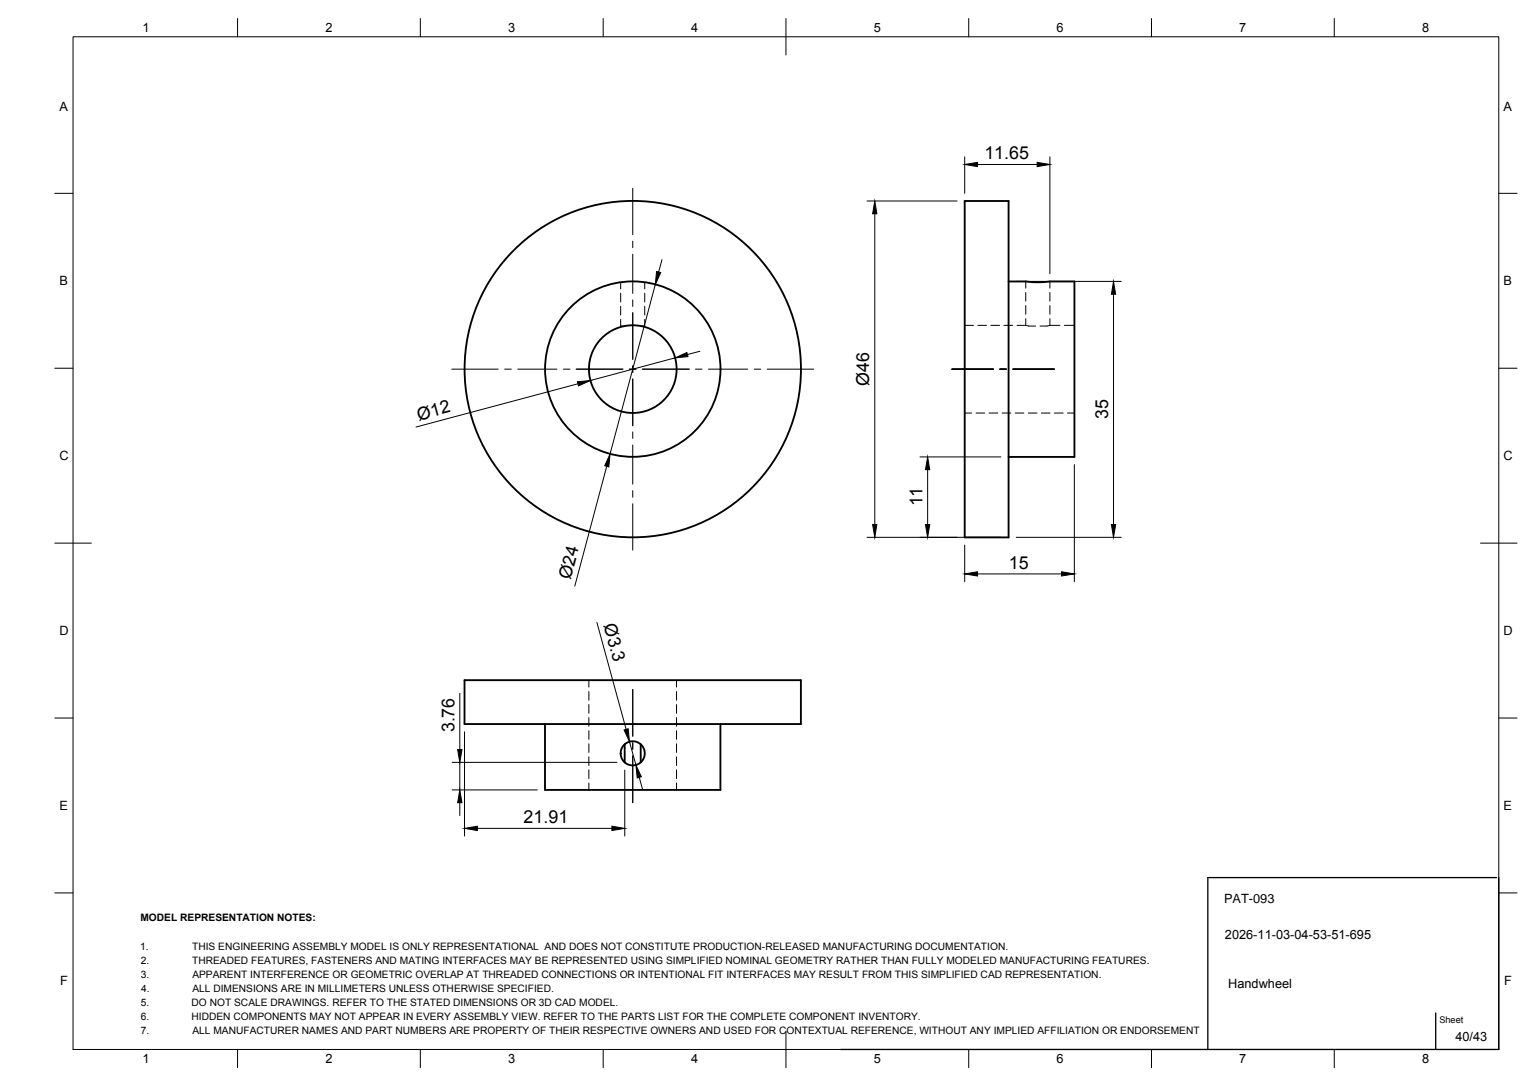
ISO-10303-21;
HEADER;
/* Generated by software containing ST-Developer
 * from STEP Tools, Inc. (www.steptools.com) 
 */

FILE_DESCRIPTION(
/* description */ ('Self-centering screw clamp'),
/* implementation_level */ '2;1');

FILE_NAME(
/* name */ 'Handwheel.step',
/* time_stamp */ '2026-10-28T03:25:31-07:00',
/* author */ (''),
/* organization */ (''),
/* preprocessor_version */ 'ST-DEVELOPER v20.2',
/* originating_system */ 'Autodesk Translation Framework v15.17.0.0',
/* authorisation */ '');

FILE_SCHEMA (('AUTOMOTIVE_DESIGN { 1 0 10303 214 3 1 1 }'));
ENDSEC;

DATA;
#10=MECHANICAL_DESIGN_GEOMETRIC_PRESENTATION_REPRESENTATION('',(#666),#16799);
#528=B_SPLINE_CURVE_WITH_KNOTS('',3,(#16250,#16251,#16252,#16253,#16254,
#16255),.UNSPECIFIED.,.F.,.F.,(4,2,4),(0.635430324955929,0.687528937234027,
0.750024497760672),.UNSPECIFIED.);
#529=B_SPLINE_CURVE_WITH_KNOTS('',3,(#16259,#16260,#16261,#16262,#16263,
#16264),.UNSPECIFIED.,.F.,.F.,(4,2,4),(0.250008165920224,0.312503726446869,
0.364602338724964),.UNSPECIFIED.);
#530=B_SPLINE_CURVE_WITH_KNOTS('',3,(#16265,#16266,#16267,#16268,#16269,
#16270),.UNSPECIFIED.,.F.,.F.,(4,2,4),(0.135413993115483,0.187512605393579,
0.250008165920224),.UNSPECIFIED.);
#531=B_SPLINE_CURVE_WITH_KNOTS('',3,(#16271,#16272,#16273,#16274,#16275,
#16276),.UNSPECIFIED.,.F.,.F.,(4,2,4),(0.750024497760672,0.812520058287317,
0.864618670565415),.UNSPECIFIED.);
#532=B_SPLINE_CURVE_WITH_KNOTS('',3,(#16280,#16281,#16282,#16283,#16284,
#16285,#16286,#16287,#16288,#16289),.UNSPECIFIED.,.F.,.F.,(4,2,2,2,4),(0.,
0.0622384309821294,0.124476861964259,0.186714529331343,0.248952196698427),
 .UNSPECIFIED.);
#533=B_SPLINE_CURVE_WITH_KNOTS('',3,(#16291,#16292,#16293,#16294,#16295,
#16296,#16297,#16298,#16299,#16300),.UNSPECIFIED.,.F.,.F.,(4,2,2,2,4),(0.74685659009528,
0.809094257462364,0.871331924829448,0.933570355811577,0.995808786793707),
 .UNSPECIFIED.);
#534=B_SPLINE_CURVE_WITH_KNOTS('',3,(#16301,#16302,#16303,#16304,#16305,
#16306,#16307,#16308,#16309,#16310,#16311,#16312,#16313,#16314,#16315,#16316,
#16317,#16318),.UNSPECIFIED.,.F.,.F.,(4,2,2,2,2,2,2,2,4),(0.248952196698427,
0.311189864065511,0.373427531432595,0.435665962414724,0.497904393396853,
0.560142824378983,0.622381255361112,0.684618922728196,0.74685659009528),
 .UNSPECIFIED.);
#577=SHAPE_REPRESENTATION_RELATIONSHIP('SRR','None',#17055,#618);
#618=ADVANCED_BREP_SHAPE_REPRESENTATION('',(#713),#16793);
#666=STYLED_ITEM('',(#17319),#713);
#713=MANIFOLD_SOLID_BREP('Body1',#9118);
#1003=FACE_BOUND('',#2518,.T.);
#1004=FACE_BOUND('',#2522,.T.);
#1005=FACE_BOUND('',#2524,.T.);
#1240=PLANE('',#10557);
#1241=PLANE('',#10561);
#1242=PLANE('',#10562);
#1243=PLANE('',#10569);
#1244=PLANE('',#10570);
#1724=FACE_OUTER_BOUND('',#2513,.T.);
#1725=FACE_OUTER_BOUND('',#2514,.T.);
#1726=FACE_OUTER_BOUND('',#2515,.T.);
#1727=FACE_OUTER_BOUND('',#2516,.T.);
#1728=FACE_OUTER_BOUND('',#2517,.T.);
#1729=FACE_OUTER_BOUND('',#2519,.T.);
#1730=FACE_OUTER_BOUND('',#2520,.T.);
#1731=FACE_OUTER_BOUND('',#2521,.T.);
#1732=FACE_OUTER_BOUND('',#2523,.T.);
#2513=EDGE_LOOP('',(#8133,#8134,#8135,#8136));
#2514=EDGE_LOOP('',(#8137,#8138));
#2515=EDGE_LOOP('',(#8139,#8140,#8141,#8142,#8143,#8144,#8145,#8146,#8147,
#8148,#8149));
#2516=EDGE_LOOP('',(#8150,#8151));
#2517=EDGE_LOOP('',(#8152));
#2518=EDGE_LOOP('',(#8153));
#2519=EDGE_LOOP('',(#8154,#8155,#8156,#8157,#8158,#8159,#8160,#8161,#8162,
#8163,#8164,#8165));
#2520=EDGE_LOOP('',(#8166,#8167,#8168,#8169,#8170,#8171,#8172,#8173,#8174));
#2521=EDGE_LOOP('',(#8175));
#2522=EDGE_LOOP('',(#8176));
#2523=EDGE_LOOP('',(#8177));
#2524=EDGE_LOOP('',(#8178));
#3086=LINE('',#16240,#3659);
#3087=LINE('',#16245,#3660);
#3088=LINE('',#16278,#3661);
#3089=LINE('',#16320,#3662);
#3090=LINE('',#16327,#3663);
#3091=LINE('',#16329,#3664);
#3092=LINE('',#16334,#3665);
#3093=LINE('',#16335,#3666);
#3659=VECTOR('',#13219,2.3);
#3660=VECTOR('',#13224,1.);
#3661=VECTOR('',#13231,0.164999999999999);
#3662=VECTOR('',#13234,1.);
#3663=VECTOR('',#13243,0.6);
#3664=VECTOR('',#13244,0.6);
#3665=VECTOR('',#13251,1.2);
#3666=VECTOR('',#13252,1.2);
#4199=CIRCLE('',#10555,2.3);
#4200=CIRCLE('',#10556,2.3);
#4201=CIRCLE('',#10558,0.164999999999999);
#4202=CIRCLE('',#10560,0.164999999999999);
#4203=CIRCLE('',#10563,1.2);
#4204=CIRCLE('',#10565,0.6);
#4205=CIRCLE('',#10566,0.6);
#4206=CIRCLE('',#10568,1.2);
#4904=VERTEX_POINT('',#16237);
#4905=VERTEX_POINT('',#16239);
#4906=VERTEX_POINT('',#16243);
#4907=VERTEX_POINT('',#16244);
#4908=VERTEX_POINT('',#16248);
#4909=VERTEX_POINT('',#16249);
#4910=VERTEX_POINT('',#16256);
#4911=VERTEX_POINT('',#16258);
#4912=VERTEX_POINT('',#16277);
#4913=VERTEX_POINT('',#16279);
#4914=VERTEX_POINT('',#16290);
#4915=VERTEX_POINT('',#16322);
#4916=VERTEX_POINT('',#16325);
#4917=VERTEX_POINT('',#16328);
#4918=VERTEX_POINT('',#16332);
#5991=EDGE_CURVE('',#4904,#4904,#4199,.T.);
#5992=EDGE_CURVE('',#4904,#4905,#3086,.T.);
#5993=EDGE_CURVE('',#4905,#4905,#4200,.T.);
#5994=EDGE_CURVE('',#4906,#4907,#3087,.T.);
#5995=EDGE_CURVE('',#4906,#4907,#4201,.T.);
#5996=EDGE_CURVE('',#4908,#4909,#528,.T.);
#5997=EDGE_CURVE('',#4910,#4908,#4202,.T.);
#5998=EDGE_CURVE('',#4911,#4910,#529,.T.);
#5999=EDGE_CURVE('',#4907,#4911,#530,.T.);
#6000=EDGE_CURVE('',#4909,#4906,#531,.T.);
#6001=EDGE_CURVE('',#4909,#4912,#3088,.T.);
#6002=EDGE_CURVE('',#4913,#4912,#532,.T.);
#6003=EDGE_CURVE('',#4914,#4913,#533,.T.);
#6004=EDGE_CURVE('',#4912,#4914,#534,.T.);
#6005=EDGE_CURVE('',#4910,#4908,#3089,.T.);
#6006=EDGE_CURVE('',#4915,#4915,#4203,.T.);
#6007=EDGE_CURVE('',#4916,#4916,#4204,.T.);
#6008=EDGE_CURVE('',#4916,#4911,#3090,.T.);
#6009=EDGE_CURVE('',#4909,#4917,#3091,.T.);
#6010=EDGE_CURVE('',#4917,#4917,#4205,.T.);
#6011=EDGE_CURVE('',#4918,#4918,#4206,.T.);
#6012=EDGE_CURVE('',#4918,#4914,#3092,.T.);
#6013=EDGE_CURVE('',#4912,#4915,#3093,.T.);
#8133=ORIENTED_EDGE('',*,*,#5991,.F.);
#8134=ORIENTED_EDGE('',*,*,#5992,.T.);
#8135=ORIENTED_EDGE('',*,*,#5993,.F.);
#8136=ORIENTED_EDGE('',*,*,#5992,.F.);
#8137=ORIENTED_EDGE('',*,*,#5994,.F.);
#8138=ORIENTED_EDGE('',*,*,#5995,.T.);
#8139=ORIENTED_EDGE('',*,*,#5996,.F.);
#8140=ORIENTED_EDGE('',*,*,#5997,.F.);
#8141=ORIENTED_EDGE('',*,*,#5998,.F.);
#8142=ORIENTED_EDGE('',*,*,#5999,.F.);
#8143=ORIENTED_EDGE('',*,*,#5995,.F.);
#8144=ORIENTED_EDGE('',*,*,#6000,.F.);
#8145=ORIENTED_EDGE('',*,*,#6001,.T.);
#8146=ORIENTED_EDGE('',*,*,#6002,.F.);
#8147=ORIENTED_EDGE('',*,*,#6003,.F.);
#8148=ORIENTED_EDGE('',*,*,#6004,.F.);
#8149=ORIENTED_EDGE('',*,*,#6001,.F.);
#8150=ORIENTED_EDGE('',*,*,#6005,.F.);
#8151=ORIENTED_EDGE('',*,*,#5997,.T.);
#8152=ORIENTED_EDGE('',*,*,#5993,.T.);
#8153=ORIENTED_EDGE('',*,*,#6006,.F.);
#8154=ORIENTED_EDGE('',*,*,#6007,.F.);
#8155=ORIENTED_EDGE('',*,*,#6008,.T.);
#8156=ORIENTED_EDGE('',*,*,#5998,.T.);
#8157=ORIENTED_EDGE('',*,*,#6005,.T.);
#8158=ORIENTED_EDGE('',*,*,#5996,.T.);
#8159=ORIENTED_EDGE('',*,*,#6009,.T.);
#8160=ORIENTED_EDGE('',*,*,#6010,.T.);
#8161=ORIENTED_EDGE('',*,*,#6009,.F.);
#8162=ORIENTED_EDGE('',*,*,#6000,.T.);
#8163=ORIENTED_EDGE('',*,*,#5994,.T.);
#8164=ORIENTED_EDGE('',*,*,#5999,.T.);
#8165=ORIENTED_EDGE('',*,*,#6008,.F.);
#8166=ORIENTED_EDGE('',*,*,#6011,.F.);
#8167=ORIENTED_EDGE('',*,*,#6012,.T.);
#8168=ORIENTED_EDGE('',*,*,#6003,.T.);
#8169=ORIENTED_EDGE('',*,*,#6002,.T.);
#8170=ORIENTED_EDGE('',*,*,#6013,.T.);
#8171=ORIENTED_EDGE('',*,*,#6006,.T.);
#8172=ORIENTED_EDGE('',*,*,#6013,.F.);
#8173=ORIENTED_EDGE('',*,*,#6004,.T.);
#8174=ORIENTED_EDGE('',*,*,#6012,.F.);
#8175=ORIENTED_EDGE('',*,*,#6011,.T.);
#8176=ORIENTED_EDGE('',*,*,#6007,.T.);
#8177=ORIENTED_EDGE('',*,*,#5991,.T.);
#8178=ORIENTED_EDGE('',*,*,#6010,.F.);
#8557=CYLINDRICAL_SURFACE('',#10554,2.3);
#8558=CYLINDRICAL_SURFACE('',#10559,0.164999999999999);
#8559=CYLINDRICAL_SURFACE('',#10564,0.6);
#8560=CYLINDRICAL_SURFACE('',#10567,1.2);
#9022=ADVANCED_FACE('',(#1724),#8557,.T.);
#9023=ADVANCED_FACE('',(#1725),#1240,.T.);
#9024=ADVANCED_FACE('',(#1726),#8558,.F.);
#9025=ADVANCED_FACE('',(#1727),#1241,.T.);
#9026=ADVANCED_FACE('',(#1728,#1003),#1242,.T.);
#9027=ADVANCED_FACE('',(#1729),#8559,.F.);
#9028=ADVANCED_FACE('',(#1730),#8560,.T.);
#9029=ADVANCED_FACE('',(#1731,#1004),#1243,.T.);
#9030=ADVANCED_FACE('',(#1732,#1005),#1244,.F.);
#9118=CLOSED_SHELL('',(#9022,#9023,#9024,#9025,#9026,#9027,#9028,#9029,
#9030));
#10553=AXIS2_PLACEMENT_3D('',#16235,#13213,#13214);
#10554=AXIS2_PLACEMENT_3D('',#16236,#13215,#13216);
#10555=AXIS2_PLACEMENT_3D('',#16238,#13217,#13218);
#10556=AXIS2_PLACEMENT_3D('',#16241,#13220,#13221);
#10557=AXIS2_PLACEMENT_3D('',#16242,#13222,#13223);
#10558=AXIS2_PLACEMENT_3D('',#16246,#13225,#13226);
#10559=AXIS2_PLACEMENT_3D('',#16247,#13227,#13228);
#10560=AXIS2_PLACEMENT_3D('',#16257,#13229,#13230);
#10561=AXIS2_PLACEMENT_3D('',#16319,#13232,#13233);
#10562=AXIS2_PLACEMENT_3D('',#16321,#13235,#13236);
#10563=AXIS2_PLACEMENT_3D('',#16323,#13237,#13238);
#10564=AXIS2_PLACEMENT_3D('',#16324,#13239,#13240);
#10565=AXIS2_PLACEMENT_3D('',#16326,#13241,#13242);
#10566=AXIS2_PLACEMENT_3D('',#16330,#13245,#13246);
#10567=AXIS2_PLACEMENT_3D('',#16331,#13247,#13248);
#10568=AXIS2_PLACEMENT_3D('',#16333,#13249,#13250);
#10569=AXIS2_PLACEMENT_3D('',#16336,#13253,#13254);
#10570=AXIS2_PLACEMENT_3D('',#16337,#13255,#13256);
#13213=DIRECTION('axis',(0.,0.,1.));
#13214=DIRECTION('refdir',(1.,0.,0.));
#13215=DIRECTION('center_axis',(1.,0.,0.));
#13216=DIRECTION('ref_axis',(0.,0.,-1.));
#13217=DIRECTION('center_axis',(-1.,0.,0.));
#13218=DIRECTION('ref_axis',(0.,0.,-1.));
#13219=DIRECTION('',(1.,0.,0.));
#13220=DIRECTION('center_axis',(1.,0.,0.));
#13221=DIRECTION('ref_axis',(0.,0.,-1.));
#13222=DIRECTION('center_axis',(0.,0.,1.));
#13223=DIRECTION('ref_axis',(1.,0.,0.));
#13224=DIRECTION('',(1.,0.,0.));
#13225=DIRECTION('center_axis',(0.,0.,1.));
#13226=DIRECTION('ref_axis',(1.,0.,0.));
#13227=DIRECTION('center_axis',(0.,0.,1.));
#13228=DIRECTION('ref_axis',(1.,0.,0.));
#13229=DIRECTION('center_axis',(0.,0.,1.));
#13230=DIRECTION('ref_axis',(1.,0.,0.));
#13231=DIRECTION('',(0.,0.,1.));
#13232=DIRECTION('center_axis',(0.,0.,1.));
#13233=DIRECTION('ref_axis',(1.,0.,0.));
#13234=DIRECTION('',(-1.,0.,0.));
#13235=DIRECTION('center_axis',(1.,0.,0.));
#13236=DIRECTION('ref_axis',(0.,0.,-1.));
#13237=DIRECTION('center_axis',(1.,0.,0.));
#13238=DIRECTION('ref_axis',(0.,0.,-1.));
#13239=DIRECTION('center_axis',(1.,0.,0.));
#13240=DIRECTION('ref_axis',(0.,0.,-1.));
#13241=DIRECTION('center_axis',(-1.,0.,0.));
#13242=DIRECTION('ref_axis',(0.,0.,-1.));
#13243=DIRECTION('',(-1.,0.,0.));
#13244=DIRECTION('',(-1.,0.,0.));
#13245=DIRECTION('center_axis',(-1.,0.,0.));
#13246=DIRECTION('ref_axis',(0.,0.,-1.));
#13247=DIRECTION('center_axis',(1.,0.,0.));
#13248=DIRECTION('ref_axis',(0.,0.,-1.));
#13249=DIRECTION('center_axis',(1.,0.,0.));
#13250=DIRECTION('ref_axis',(0.,0.,-1.));
#13251=DIRECTION('',(-1.,0.,0.));
#13252=DIRECTION('',(-1.,0.,0.));
#13253=DIRECTION('center_axis',(1.,0.,0.));
#13254=DIRECTION('ref_axis',(0.,0.,-1.));
#13255=DIRECTION('center_axis',(1.,0.,0.));
#13256=DIRECTION('ref_axis',(0.,0.,-1.));
#16235=CARTESIAN_POINT('',(0.,0.,0.));
#16236=CARTESIAN_POINT('Origin',(-15.1,0.,4.));
#16237=CARTESIAN_POINT('',(-15.,2.81668763803891E-16,6.3));
#16238=CARTESIAN_POINT('Origin',(-15.,0.,4.));
#16239=CARTESIAN_POINT('',(-14.4,-2.81668763803891E-16,6.3));
#16240=CARTESIAN_POINT('',(-15.1,-2.81668763803891E-16,6.3));
#16241=CARTESIAN_POINT('Origin',(-14.4,0.,4.));
#16242=CARTESIAN_POINT('Origin',(-14.,0.,4.59));
#16243=CARTESIAN_POINT('',(-14.1237941840314,-0.109087121146358,4.59));
#16244=CARTESIAN_POINT('',(-13.8762058159686,-0.109087121146358,4.59));
#16245=CARTESIAN_POINT('',(-15.,-0.109087121146358,4.59));
#16246=CARTESIAN_POINT('Origin',(-14.,0.,4.59));
#16247=CARTESIAN_POINT('Origin',(-14.,0.,4.59));
#16248=CARTESIAN_POINT('',(-14.1237941840314,0.109087121146358,4.59));
#16249=CARTESIAN_POINT('',(-14.165,1.24480690947329E-17,4.6));
#16250=CARTESIAN_POINT('Ctrl Pts',(-14.1237941840314,0.109087121146359,
4.59));
#16251=CARTESIAN_POINT('Ctrl Pts',(-14.1353991351895,0.0959175971526122,
4.59243495840567));
#16252=CARTESIAN_POINT('Ctrl Pts',(-14.1453456436582,0.080223449437719,
4.59485638705045));
#16253=CARTESIAN_POINT('Ctrl Pts',(-14.160814864634,0.04298016596019,4.59880705606552));
#16254=CARTESIAN_POINT('Ctrl Pts',(-14.165,0.0208318535088818,4.6));
#16255=CARTESIAN_POINT('Ctrl Pts',(-14.165,2.77555756156289E-17,4.6));
#16256=CARTESIAN_POINT('',(-13.8762058159686,0.109087121146358,4.59));
#16257=CARTESIAN_POINT('Origin',(-14.,0.,4.59));
#16258=CARTESIAN_POINT('',(-13.835,-8.98382835879169E-18,4.6));
#16259=CARTESIAN_POINT('Ctrl Pts',(-13.835,-2.08166817117217E-17,4.6));
#16260=CARTESIAN_POINT('Ctrl Pts',(-13.835,0.0208318535088817,4.6));
#16261=CARTESIAN_POINT('Ctrl Pts',(-13.839185135366,0.0429801659601899,
4.59880705606552));
#16262=CARTESIAN_POINT('Ctrl Pts',(-13.8546543563418,0.0802234494377183,
4.59485638705045));
#16263=CARTESIAN_POINT('Ctrl Pts',(-13.8646008648105,0.0959175971526114,
4.59243495840567));
#16264=CARTESIAN_POINT('Ctrl Pts',(-13.8762058159686,0.109087121146357,
4.59));
#16265=CARTESIAN_POINT('Ctrl Pts',(-13.8762058159686,-0.109087121146357,
4.59));
#16266=CARTESIAN_POINT('Ctrl Pts',(-13.8646008648105,-0.0959175971526111,
4.59243495840567));
#16267=CARTESIAN_POINT('Ctrl Pts',(-13.8546543563418,-0.0802234494377185,
4.59485638705045));
#16268=CARTESIAN_POINT('Ctrl Pts',(-13.839185135366,-0.0429801659601899,
4.59880705606552));
#16269=CARTESIAN_POINT('Ctrl Pts',(-13.835,-0.0208318535088816,4.6));
#16270=CARTESIAN_POINT('Ctrl Pts',(-13.835,1.31838984174237E-16,4.6));
#16271=CARTESIAN_POINT('Ctrl Pts',(-14.165,-6.93889390390723E-18,4.6));
#16272=CARTESIAN_POINT('Ctrl Pts',(-14.165,-0.0208318535088817,4.6));
#16273=CARTESIAN_POINT('Ctrl Pts',(-14.160814864634,-0.04298016596019,4.59880705606552));
#16274=CARTESIAN_POINT('Ctrl Pts',(-14.1453456436582,-0.0802234494377193,
4.59485638705045));
#16275=CARTESIAN_POINT('Ctrl Pts',(-14.1353991351895,-0.0959175971526121,
4.59243495840567));
#16276=CARTESIAN_POINT('Ctrl Pts',(-14.1237941840314,-0.109087121146359,
4.59));
#16277=CARTESIAN_POINT('',(-14.165,-2.02066721859312E-17,5.2));
#16278=CARTESIAN_POINT('',(-14.165,-2.02066721859312E-17,4.59));
#16279=CARTESIAN_POINT('',(-14.,-0.164999999999999,5.18860212013945));
#16280=CARTESIAN_POINT('Ctrl Pts',(-14.,-0.164999999999999,5.18860212013945));
#16281=CARTESIAN_POINT('Ctrl Pts',(-14.0207461436607,-0.164999999999999,
5.18860212013945));
#16282=CARTESIAN_POINT('Ctrl Pts',(-14.0428569170208,-0.160848489718829,
5.18920136323583));
#16283=CARTESIAN_POINT('Ctrl Pts',(-14.0835015842248,-0.144001521209443,
5.19135875380323));
#16284=CARTESIAN_POINT('Ctrl Pts',(-14.1020377548452,-0.131307482946398,
5.19288497691659));
#16285=CARTESIAN_POINT('Ctrl Pts',(-14.1313073033885,-0.102037934403068,
5.19574431960517));
#16286=CARTESIAN_POINT('Ctrl Pts',(-14.1440014824454,-0.0835016860163233,
5.1972642227448));
#16287=CARTESIAN_POINT('Ctrl Pts',(-14.1608485537388,-0.0428567542973034,
5.19940712405299));
#16288=CARTESIAN_POINT('Ctrl Pts',(-14.165,-0.0207458891223613,5.2));
#16289=CARTESIAN_POINT('Ctrl Pts',(-14.165,2.77555756156289E-17,5.2));
#16290=CARTESIAN_POINT('',(-13.835,-6.30704670929804E-17,5.2));
#16291=CARTESIAN_POINT('Ctrl Pts',(-13.835,3.46944695195361E-17,5.2));
#16292=CARTESIAN_POINT('Ctrl Pts',(-13.835,-0.0207458891223613,5.2));
#16293=CARTESIAN_POINT('Ctrl Pts',(-13.8391514462612,-0.0428567542973019,
5.19940712405299));
#16294=CARTESIAN_POINT('Ctrl Pts',(-13.8559985175546,-0.083501686016322,
5.1972642227448));
#16295=CARTESIAN_POINT('Ctrl Pts',(-13.8686926966115,-0.102037934403068,
5.19574431960517));
#16296=CARTESIAN_POINT('Ctrl Pts',(-13.8979622451548,-0.131307482946398,
5.19288497691659));
#16297=CARTESIAN_POINT('Ctrl Pts',(-13.9164984157752,-0.144001521209443,
5.19135875380323));
#16298=CARTESIAN_POINT('Ctrl Pts',(-13.9571430829792,-0.160848489718829,
5.18920136323583));
#16299=CARTESIAN_POINT('Ctrl Pts',(-13.9792538563393,-0.164999999999999,
5.18860212013945));
#16300=CARTESIAN_POINT('Ctrl Pts',(-14.,-0.164999999999999,5.18860212013945));
#16301=CARTESIAN_POINT('Ctrl Pts',(-14.165,2.08166817117217E-17,5.2));
#16302=CARTESIAN_POINT('Ctrl Pts',(-14.165,0.0207458891223613,5.2));
#16303=CARTESIAN_POINT('Ctrl Pts',(-14.1608485537388,0.042856754297302,
5.19940712405299));
#16304=CARTESIAN_POINT('Ctrl Pts',(-14.1440014824454,0.083501686016322,
5.1972642227448));
#16305=CARTESIAN_POINT('Ctrl Pts',(-14.1313073033885,0.102037934403068,
5.19574431960517));
#16306=CARTESIAN_POINT('Ctrl Pts',(-14.1020377548452,0.131307482946398,
5.19288497691659));
#16307=CARTESIAN_POINT('Ctrl Pts',(-14.0835015842248,0.144001521209443,
5.19135875380323));
#16308=CARTESIAN_POINT('Ctrl Pts',(-14.0428569170208,0.160848489718829,
5.18920136323583));
#16309=CARTESIAN_POINT('Ctrl Pts',(-14.0207461436607,0.164999999999999,
5.18860212013945));
#16310=CARTESIAN_POINT('Ctrl Pts',(-13.9792538563393,0.164999999999999,
5.18860212013945));
#16311=CARTESIAN_POINT('Ctrl Pts',(-13.9571430829792,0.160848489718829,
5.18920136323583));
#16312=CARTESIAN_POINT('Ctrl Pts',(-13.9164984157752,0.144001521209443,
5.19135875380323));
#16313=CARTESIAN_POINT('Ctrl Pts',(-13.8979622451548,0.131307482946398,
5.19288497691659));
#16314=CARTESIAN_POINT('Ctrl Pts',(-13.8686926966115,0.102037934403068,
5.19574431960517));
#16315=CARTESIAN_POINT('Ctrl Pts',(-13.8559985175546,0.083501686016322,
5.1972642227448));
#16316=CARTESIAN_POINT('Ctrl Pts',(-13.8391514462612,0.042856754297302,
5.19940712405299));
#16317=CARTESIAN_POINT('Ctrl Pts',(-13.835,0.0207458891223614,5.2));
#16318=CARTESIAN_POINT('Ctrl Pts',(-13.835,4.85722573273506E-17,5.2));
#16319=CARTESIAN_POINT('Origin',(-14.,0.,4.59));
#16320=CARTESIAN_POINT('',(-15.,0.109087121146358,4.59));
#16321=CARTESIAN_POINT('Origin',(-14.4,0.,4.));
#16322=CARTESIAN_POINT('',(-14.4,-1.46957615897682E-16,5.2));
#16323=CARTESIAN_POINT('Origin',(-14.4,0.,4.));
#16324=CARTESIAN_POINT('Origin',(-15.,0.,4.));
#16325=CARTESIAN_POINT('',(-13.5,-7.34788079488412E-17,4.6));
#16326=CARTESIAN_POINT('Origin',(-13.5,0.,4.));
#16327=CARTESIAN_POINT('',(-15.,-7.34788079488412E-17,4.6));
#16328=CARTESIAN_POINT('',(-15.,-7.34788079488412E-17,4.6));
#16329=CARTESIAN_POINT('',(-15.,-7.34788079488412E-17,4.6));
#16330=CARTESIAN_POINT('Origin',(-15.,0.,4.));
#16331=CARTESIAN_POINT('Origin',(-15.,0.,4.));
#16332=CARTESIAN_POINT('',(-13.5,-1.46957615897682E-16,5.2));
#16333=CARTESIAN_POINT('Origin',(-13.5,0.,4.));
#16334=CARTESIAN_POINT('',(-15.,-1.46957615897682E-16,5.2));
#16335=CARTESIAN_POINT('',(-15.,-1.46957615897682E-16,5.2));
#16336=CARTESIAN_POINT('Origin',(-13.5,0.,4.));
#16337=CARTESIAN_POINT('Origin',(-15.,0.,4.));
#16744=UNCERTAINTY_MEASURE_WITH_UNIT(LENGTH_MEASURE(0.001),#16800,
'DISTANCE_ACCURACY_VALUE',
'Maximum model space distance between geometric entities at asserted c
onnectivities');
#16750=UNCERTAINTY_MEASURE_WITH_UNIT(LENGTH_MEASURE(0.001),#16800,
'DISTANCE_ACCURACY_VALUE',
'Maximum model space distance between geometric entities at asserted c
onnectivities');
#16793=(
GEOMETRIC_REPRESENTATION_CONTEXT(3)
GLOBAL_UNCERTAINTY_ASSIGNED_CONTEXT((#16744))
GLOBAL_UNIT_ASSIGNED_CONTEXT((#16800,#16802,#16803))
REPRESENTATION_CONTEXT('','3D')
);
#16799=(
GEOMETRIC_REPRESENTATION_CONTEXT(3)
GLOBAL_UNCERTAINTY_ASSIGNED_CONTEXT((#16750))
GLOBAL_UNIT_ASSIGNED_CONTEXT((#16800,#16802,#16803))
REPRESENTATION_CONTEXT('','3D')
);
#16800=(
LENGTH_UNIT()
NAMED_UNIT(*)
SI_UNIT(.CENTI.,.METRE.)
);
#16802=(
NAMED_UNIT(*)
PLANE_ANGLE_UNIT()
SI_UNIT($,.RADIAN.)
);
#16803=(
NAMED_UNIT(*)
SI_UNIT($,.STERADIAN.)
SOLID_ANGLE_UNIT()
);
#16846=SHAPE_DEFINITION_REPRESENTATION(#16901,#17055);
#16901=PRODUCT_DEFINITION_SHAPE('',$,#17104);
#17055=SHAPE_REPRESENTATION('',(#10553),#16793);
#17061=PRODUCT_DEFINITION_CONTEXT('part definition',#17207,'design');
#17104=PRODUCT_DEFINITION('Handwheel','Handwheel',#17152,#17061);
#17152=PRODUCT_DEFINITION_FORMATION('',$,#17251);
#17207=APPLICATION_CONTEXT(
'Core Data for Automotive Mechanical Design Process');
#17208=PRODUCT_CONTEXT('part definition',#17207,'mechanical');
#17251=PRODUCT('Handwheel','Handwheel','Handwheel',(#17208));
#17313=COLOUR_RGB('Sky Blue',0.24,0.69,0.87);
#17314=FILL_AREA_STYLE_COLOUR('',#17313);
#17315=FILL_AREA_STYLE('',(#17314));
#17316=SURFACE_STYLE_FILL_AREA(#17315);
#17317=SURFACE_SIDE_STYLE('',(#17316));
#17318=SURFACE_STYLE_USAGE(.BOTH.,#17317);
#17319=PRESENTATION_STYLE_ASSIGNMENT((#17318));
ENDSEC;
END-ISO-10303-21;
